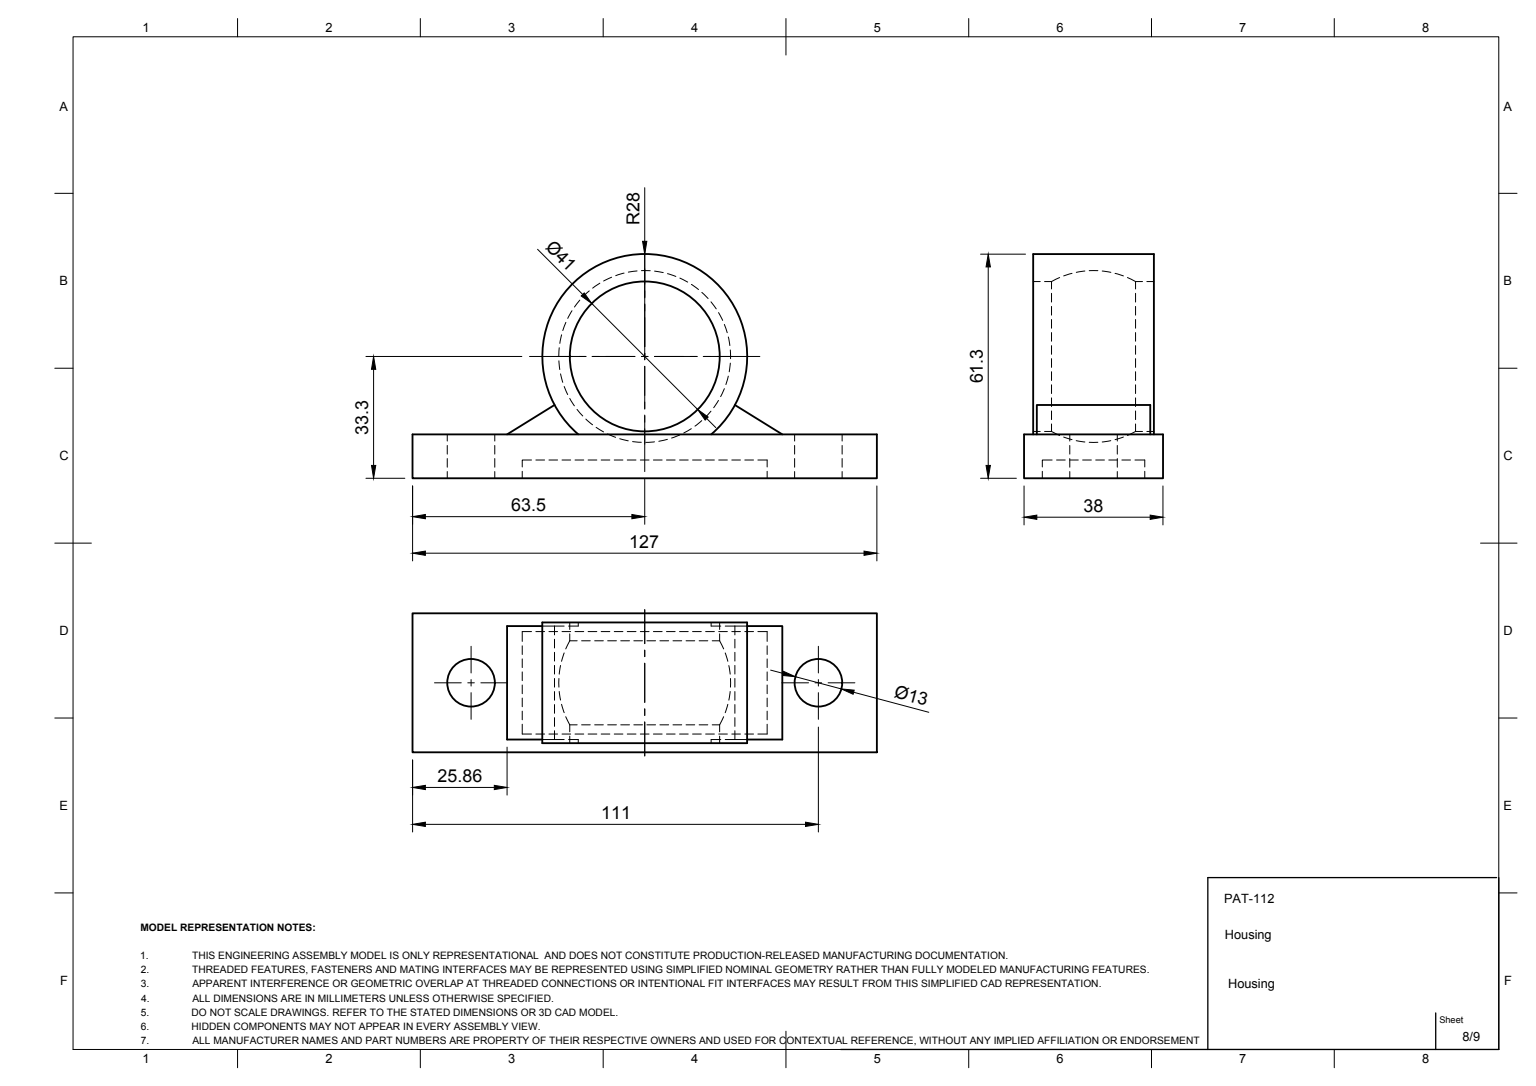
ISO-10303-21;
HEADER;
/* Generated by software containing ST-Developer
 * from STEP Tools, Inc. (www.steptools.com) 
 */

FILE_DESCRIPTION(
/* description */ ('PAT-112'),
/* implementation_level */ '2;1');

FILE_NAME(
/* name */ 'Housing.step',
/* time_stamp */ '2026-11-15T15:25:42-08:00',
/* author */ (''),
/* organization */ (''),
/* preprocessor_version */ 'ST-DEVELOPER v20.2',
/* originating_system */ 'Autodesk Translation Framework v15.17.0.0',
/* authorisation */ '');

FILE_SCHEMA (('AUTOMOTIVE_DESIGN { 1 0 10303 214 3 1 1 }'));
ENDSEC;

DATA;
#10=MECHANICAL_DESIGN_GEOMETRIC_PRESENTATION_REPRESENTATION('',(#106),#2277);
#89=SPHERICAL_SURFACE('',#1376,2.35);
#92=SHAPE_REPRESENTATION_RELATIONSHIP('SRR','None',#2321,#99);
#99=ADVANCED_BREP_SHAPE_REPRESENTATION('',(#114),#2271);
#106=STYLED_ITEM('',(#2368),#114);
#114=MANIFOLD_SOLID_BREP('Body1',#1258);
#124=FACE_BOUND('',#295,.T.);
#125=FACE_BOUND('',#296,.T.);
#126=FACE_BOUND('',#304,.T.);
#127=FACE_BOUND('',#305,.T.);
#128=FACE_BOUND('',#306,.T.);
#129=FACE_BOUND('',#309,.T.);
#130=FACE_BOUND('',#311,.T.);
#131=FACE_BOUND('',#324,.T.);
#132=FACE_BOUND('',#325,.T.);
#133=FACE_BOUND('',#326,.T.);
#156=PLANE('',#1378);
#157=PLANE('',#1380);
#158=PLANE('',#1382);
#159=PLANE('',#1384);
#160=PLANE('',#1385);
#161=PLANE('',#1387);
#162=PLANE('',#1388);
#163=PLANE('',#1394);
#164=PLANE('',#1395);
#165=PLANE('',#1396);
#166=PLANE('',#1397);
#167=PLANE('',#1398);
#168=PLANE('',#1399);
#169=PLANE('',#1400);
#170=PLANE('',#1405);
#171=PLANE('',#1406);
#172=PLANE('',#1407);
#173=PLANE('',#1408);
#174=PLANE('',#1409);
#211=FACE_OUTER_BOUND('',#292,.T.);
#212=FACE_OUTER_BOUND('',#293,.T.);
#213=FACE_OUTER_BOUND('',#294,.T.);
#214=FACE_OUTER_BOUND('',#297,.T.);
#215=FACE_OUTER_BOUND('',#298,.T.);
#216=FACE_OUTER_BOUND('',#299,.T.);
#217=FACE_OUTER_BOUND('',#300,.T.);
#218=FACE_OUTER_BOUND('',#301,.T.);
#219=FACE_OUTER_BOUND('',#302,.T.);
#220=FACE_OUTER_BOUND('',#303,.T.);
#221=FACE_OUTER_BOUND('',#307,.T.);
#222=FACE_OUTER_BOUND('',#308,.T.);
#223=FACE_OUTER_BOUND('',#310,.T.);
#224=FACE_OUTER_BOUND('',#312,.T.);
#225=FACE_OUTER_BOUND('',#313,.T.);
#226=FACE_OUTER_BOUND('',#314,.T.);
#227=FACE_OUTER_BOUND('',#315,.T.);
#228=FACE_OUTER_BOUND('',#316,.T.);
#229=FACE_OUTER_BOUND('',#317,.T.);
#230=FACE_OUTER_BOUND('',#318,.T.);
#231=FACE_OUTER_BOUND('',#319,.T.);
#232=FACE_OUTER_BOUND('',#320,.T.);
#233=FACE_OUTER_BOUND('',#321,.T.);
#234=FACE_OUTER_BOUND('',#322,.T.);
#235=FACE_OUTER_BOUND('',#323,.T.);
#292=EDGE_LOOP('',(#914,#915,#916,#917));
#293=EDGE_LOOP('',(#918,#919,#920,#921));
#294=EDGE_LOOP('',(#922,#923));
#295=EDGE_LOOP('',(#924));
#296=EDGE_LOOP('',(#925));
#297=EDGE_LOOP('',(#926,#927,#928));
#298=EDGE_LOOP('',(#929,#930,#931));
#299=EDGE_LOOP('',(#932,#933,#934));
#300=EDGE_LOOP('',(#935,#936,#937,#938));
#301=EDGE_LOOP('',(#939,#940,#941));
#302=EDGE_LOOP('',(#942,#943,#944,#945));
#303=EDGE_LOOP('',(#946,#947,#948,#949));
#304=EDGE_LOOP('',(#950));
#305=EDGE_LOOP('',(#951));
#306=EDGE_LOOP('',(#952,#953,#954,#955,#956,#957,#958,#959,#960,#961,#962,
#963));
#307=EDGE_LOOP('',(#964,#965,#966,#967,#968,#969,#970,#971,#972,#973,#974,
#975));
#308=EDGE_LOOP('',(#976,#977));
#309=EDGE_LOOP('',(#978));
#310=EDGE_LOOP('',(#979,#980));
#311=EDGE_LOOP('',(#981));
#312=EDGE_LOOP('',(#982,#983,#984,#985));
#313=EDGE_LOOP('',(#986,#987,#988,#989));
#314=EDGE_LOOP('',(#990,#991,#992,#993));
#315=EDGE_LOOP('',(#994,#995,#996,#997));
#316=EDGE_LOOP('',(#998,#999,#1000,#1001));
#317=EDGE_LOOP('',(#1002,#1003,#1004,#1005));
#318=EDGE_LOOP('',(#1006,#1007,#1008,#1009));
#319=EDGE_LOOP('',(#1010,#1011,#1012,#1013));
#320=EDGE_LOOP('',(#1014,#1015,#1016,#1017));
#321=EDGE_LOOP('',(#1018,#1019,#1020,#1021));
#322=EDGE_LOOP('',(#1022,#1023,#1024,#1025));
#323=EDGE_LOOP('',(#1026,#1027,#1028,#1029));
#324=EDGE_LOOP('',(#1030,#1031,#1032,#1033));
#325=EDGE_LOOP('',(#1034));
#326=EDGE_LOOP('',(#1035));
#393=LINE('',#1969,#488);
#394=LINE('',#1975,#489);
#395=LINE('',#1984,#490);
#396=LINE('',#1986,#491);
#397=LINE('',#1991,#492);
#398=LINE('',#1994,#493);
#399=LINE('',#1998,#494);
#400=LINE('',#2001,#495);
#401=LINE('',#2003,#496);
#402=LINE('',#2004,#497);
#403=LINE('',#2008,#498);
#404=LINE('',#2010,#499);
#405=LINE('',#2013,#500);
#406=LINE('',#2014,#501);
#407=LINE('',#2018,#502);
#408=LINE('',#2020,#503);
#409=LINE('',#2022,#504);
#410=LINE('',#2023,#505);
#411=LINE('',#2029,#506);
#412=LINE('',#2031,#507);
#413=LINE('',#2032,#508);
#414=LINE('',#2034,#509);
#415=LINE('',#2036,#510);
#416=LINE('',#2037,#511);
#417=LINE('',#2046,#512);
#418=LINE('',#2048,#513);
#419=LINE('',#2050,#514);
#420=LINE('',#2051,#515);
#421=LINE('',#2054,#516);
#422=LINE('',#2056,#517);
#423=LINE('',#2057,#518);
#424=LINE('',#2060,#519);
#425=LINE('',#2062,#520);
#426=LINE('',#2063,#521);
#427=LINE('',#2065,#522);
#428=LINE('',#2066,#523);
#429=LINE('',#2071,#524);
#430=LINE('',#2075,#525);
#431=LINE('',#2079,#526);
#432=LINE('',#2080,#527);
#433=LINE('',#2081,#528);
#434=LINE('',#2084,#529);
#435=LINE('',#2085,#530);
#436=LINE('',#2088,#531);
#437=LINE('',#2089,#532);
#438=LINE('',#2091,#533);
#488=VECTOR('',#1572,2.05);
#489=VECTOR('',#1579,2.05);
#490=VECTOR('',#1588,1.);
#491=VECTOR('',#1589,1.);
#492=VECTOR('',#1594,1.);
#493=VECTOR('',#1597,1.);
#494=VECTOR('',#1600,1.);
#495=VECTOR('',#1603,1.);
#496=VECTOR('',#1606,1.);
#497=VECTOR('',#1607,1.);
#498=VECTOR('',#1610,1.);
#499=VECTOR('',#1611,1.);
#500=VECTOR('',#1616,1.);
#501=VECTOR('',#1617,1.);
#502=VECTOR('',#1620,1.);
#503=VECTOR('',#1621,1.);
#504=VECTOR('',#1622,1.);
#505=VECTOR('',#1623,1.);
#506=VECTOR('',#1628,1.);
#507=VECTOR('',#1629,1.);
#508=VECTOR('',#1630,1.);
#509=VECTOR('',#1631,1.);
#510=VECTOR('',#1632,1.);
#511=VECTOR('',#1633,1.);
#512=VECTOR('',#1646,1.);
#513=VECTOR('',#1647,1.);
#514=VECTOR('',#1648,1.);
#515=VECTOR('',#1649,1.);
#516=VECTOR('',#1652,1.);
#517=VECTOR('',#1653,1.);
#518=VECTOR('',#1654,1.);
#519=VECTOR('',#1657,1.);
#520=VECTOR('',#1658,1.);
#521=VECTOR('',#1659,1.);
#522=VECTOR('',#1662,1.);
#523=VECTOR('',#1663,1.);
#524=VECTOR('',#1670,0.65);
#525=VECTOR('',#1675,0.65);
#526=VECTOR('',#1678,1.);
#527=VECTOR('',#1679,1.);
#528=VECTOR('',#1680,1.);
#529=VECTOR('',#1683,1.);
#530=VECTOR('',#1684,1.);
#531=VECTOR('',#1687,1.);
#532=VECTOR('',#1688,1.);
#533=VECTOR('',#1691,1.);
#575=CIRCLE('',#1371,2.05);
#576=CIRCLE('',#1372,2.05);
#577=CIRCLE('',#1374,2.05);
#578=CIRCLE('',#1375,2.05);
#579=CIRCLE('',#1377,2.35);
#580=CIRCLE('',#1379,2.8);
#581=CIRCLE('',#1381,2.8);
#582=CIRCLE('',#1383,2.8);
#583=CIRCLE('',#1386,2.8);
#584=CIRCLE('',#1389,0.65);
#585=CIRCLE('',#1390,0.65);
#586=CIRCLE('',#1392,2.8);
#587=CIRCLE('',#1393,2.8);
#588=CIRCLE('',#1402,0.65);
#589=CIRCLE('',#1404,0.65);
#635=VERTEX_POINT('',#1966);
#636=VERTEX_POINT('',#1968);
#637=VERTEX_POINT('',#1972);
#638=VERTEX_POINT('',#1974);
#639=VERTEX_POINT('',#1978);
#640=VERTEX_POINT('',#1979);
#641=VERTEX_POINT('',#1982);
#642=VERTEX_POINT('',#1983);
#643=VERTEX_POINT('',#1985);
#644=VERTEX_POINT('',#1989);
#645=VERTEX_POINT('',#1990);
#646=VERTEX_POINT('',#1992);
#647=VERTEX_POINT('',#1996);
#648=VERTEX_POINT('',#1997);
#649=VERTEX_POINT('',#1999);
#650=VERTEX_POINT('',#2006);
#651=VERTEX_POINT('',#2007);
#652=VERTEX_POINT('',#2009);
#653=VERTEX_POINT('',#2016);
#654=VERTEX_POINT('',#2017);
#655=VERTEX_POINT('',#2019);
#656=VERTEX_POINT('',#2021);
#657=VERTEX_POINT('',#2024);
#658=VERTEX_POINT('',#2026);
#659=VERTEX_POINT('',#2028);
#660=VERTEX_POINT('',#2030);
#661=VERTEX_POINT('',#2033);
#662=VERTEX_POINT('',#2035);
#663=VERTEX_POINT('',#2044);
#664=VERTEX_POINT('',#2045);
#665=VERTEX_POINT('',#2047);
#666=VERTEX_POINT('',#2049);
#667=VERTEX_POINT('',#2053);
#668=VERTEX_POINT('',#2055);
#669=VERTEX_POINT('',#2059);
#670=VERTEX_POINT('',#2061);
#671=VERTEX_POINT('',#2069);
#672=VERTEX_POINT('',#2073);
#673=VERTEX_POINT('',#2077);
#674=VERTEX_POINT('',#2078);
#675=VERTEX_POINT('',#2083);
#676=VERTEX_POINT('',#2087);
#743=EDGE_CURVE('',#635,#635,#575,.T.);
#744=EDGE_CURVE('',#635,#636,#393,.T.);
#745=EDGE_CURVE('',#636,#636,#576,.T.);
#746=EDGE_CURVE('',#637,#637,#577,.T.);
#747=EDGE_CURVE('',#637,#638,#394,.T.);
#748=EDGE_CURVE('',#638,#638,#578,.T.);
#749=EDGE_CURVE('',#639,#640,#579,.T.);
#750=EDGE_CURVE('',#641,#642,#395,.T.);
#751=EDGE_CURVE('',#641,#643,#396,.T.);
#752=EDGE_CURVE('',#642,#643,#580,.T.);
#753=EDGE_CURVE('',#644,#645,#397,.T.);
#754=EDGE_CURVE('',#646,#644,#581,.T.);
#755=EDGE_CURVE('',#646,#645,#398,.T.);
#756=EDGE_CURVE('',#647,#648,#399,.T.);
#757=EDGE_CURVE('',#649,#647,#582,.T.);
#758=EDGE_CURVE('',#649,#648,#400,.T.);
#759=EDGE_CURVE('',#648,#641,#401,.T.);
#760=EDGE_CURVE('',#643,#649,#402,.T.);
#761=EDGE_CURVE('',#650,#651,#403,.T.);
#762=EDGE_CURVE('',#650,#652,#404,.T.);
#763=EDGE_CURVE('',#651,#652,#583,.T.);
#764=EDGE_CURVE('',#645,#650,#405,.T.);
#765=EDGE_CURVE('',#652,#646,#406,.T.);
#766=EDGE_CURVE('',#653,#654,#407,.T.);
#767=EDGE_CURVE('',#654,#655,#408,.T.);
#768=EDGE_CURVE('',#655,#656,#409,.T.);
#769=EDGE_CURVE('',#656,#653,#410,.T.);
#770=EDGE_CURVE('',#657,#657,#584,.T.);
#771=EDGE_CURVE('',#658,#658,#585,.T.);
#772=EDGE_CURVE('',#651,#659,#411,.T.);
#773=EDGE_CURVE('',#659,#660,#412,.T.);
#774=EDGE_CURVE('',#660,#647,#413,.T.);
#775=EDGE_CURVE('',#642,#661,#414,.T.);
#776=EDGE_CURVE('',#661,#662,#415,.T.);
#777=EDGE_CURVE('',#662,#644,#416,.T.);
#778=EDGE_CURVE('',#661,#662,#586,.T.);
#779=EDGE_CURVE('',#659,#660,#587,.T.);
#780=EDGE_CURVE('',#663,#664,#417,.T.);
#781=EDGE_CURVE('',#663,#665,#418,.T.);
#782=EDGE_CURVE('',#665,#666,#419,.T.);
#783=EDGE_CURVE('',#664,#666,#420,.T.);
#784=EDGE_CURVE('',#667,#663,#421,.T.);
#785=EDGE_CURVE('',#667,#668,#422,.T.);
#786=EDGE_CURVE('',#668,#665,#423,.T.);
#787=EDGE_CURVE('',#669,#667,#424,.T.);
#788=EDGE_CURVE('',#669,#670,#425,.T.);
#789=EDGE_CURVE('',#670,#668,#426,.T.);
#790=EDGE_CURVE('',#664,#669,#427,.T.);
#791=EDGE_CURVE('',#666,#670,#428,.T.);
#792=EDGE_CURVE('',#671,#671,#588,.T.);
#793=EDGE_CURVE('',#671,#658,#429,.T.);
#794=EDGE_CURVE('',#672,#672,#589,.T.);
#795=EDGE_CURVE('',#672,#657,#430,.T.);
#796=EDGE_CURVE('',#673,#674,#431,.T.);
#797=EDGE_CURVE('',#674,#653,#432,.T.);
#798=EDGE_CURVE('',#673,#656,#433,.T.);
#799=EDGE_CURVE('',#675,#673,#434,.T.);
#800=EDGE_CURVE('',#675,#655,#435,.T.);
#801=EDGE_CURVE('',#676,#675,#436,.T.);
#802=EDGE_CURVE('',#676,#654,#437,.T.);
#803=EDGE_CURVE('',#674,#676,#438,.T.);
#914=ORIENTED_EDGE('',*,*,#743,.F.);
#915=ORIENTED_EDGE('',*,*,#744,.T.);
#916=ORIENTED_EDGE('',*,*,#745,.F.);
#917=ORIENTED_EDGE('',*,*,#744,.F.);
#918=ORIENTED_EDGE('',*,*,#746,.F.);
#919=ORIENTED_EDGE('',*,*,#747,.T.);
#920=ORIENTED_EDGE('',*,*,#748,.F.);
#921=ORIENTED_EDGE('',*,*,#747,.F.);
#922=ORIENTED_EDGE('',*,*,#749,.T.);
#923=ORIENTED_EDGE('',*,*,#749,.F.);
#924=ORIENTED_EDGE('',*,*,#746,.T.);
#925=ORIENTED_EDGE('',*,*,#745,.T.);
#926=ORIENTED_EDGE('',*,*,#750,.F.);
#927=ORIENTED_EDGE('',*,*,#751,.T.);
#928=ORIENTED_EDGE('',*,*,#752,.F.);
#929=ORIENTED_EDGE('',*,*,#753,.F.);
#930=ORIENTED_EDGE('',*,*,#754,.F.);
#931=ORIENTED_EDGE('',*,*,#755,.T.);
#932=ORIENTED_EDGE('',*,*,#756,.F.);
#933=ORIENTED_EDGE('',*,*,#757,.F.);
#934=ORIENTED_EDGE('',*,*,#758,.T.);
#935=ORIENTED_EDGE('',*,*,#759,.F.);
#936=ORIENTED_EDGE('',*,*,#758,.F.);
#937=ORIENTED_EDGE('',*,*,#760,.F.);
#938=ORIENTED_EDGE('',*,*,#751,.F.);
#939=ORIENTED_EDGE('',*,*,#761,.F.);
#940=ORIENTED_EDGE('',*,*,#762,.T.);
#941=ORIENTED_EDGE('',*,*,#763,.F.);
#942=ORIENTED_EDGE('',*,*,#764,.F.);
#943=ORIENTED_EDGE('',*,*,#755,.F.);
#944=ORIENTED_EDGE('',*,*,#765,.F.);
#945=ORIENTED_EDGE('',*,*,#762,.F.);
#946=ORIENTED_EDGE('',*,*,#766,.T.);
#947=ORIENTED_EDGE('',*,*,#767,.T.);
#948=ORIENTED_EDGE('',*,*,#768,.T.);
#949=ORIENTED_EDGE('',*,*,#769,.T.);
#950=ORIENTED_EDGE('',*,*,#770,.T.);
#951=ORIENTED_EDGE('',*,*,#771,.T.);
#952=ORIENTED_EDGE('',*,*,#753,.T.);
#953=ORIENTED_EDGE('',*,*,#764,.T.);
#954=ORIENTED_EDGE('',*,*,#761,.T.);
#955=ORIENTED_EDGE('',*,*,#772,.T.);
#956=ORIENTED_EDGE('',*,*,#773,.T.);
#957=ORIENTED_EDGE('',*,*,#774,.T.);
#958=ORIENTED_EDGE('',*,*,#756,.T.);
#959=ORIENTED_EDGE('',*,*,#759,.T.);
#960=ORIENTED_EDGE('',*,*,#750,.T.);
#961=ORIENTED_EDGE('',*,*,#775,.T.);
#962=ORIENTED_EDGE('',*,*,#776,.T.);
#963=ORIENTED_EDGE('',*,*,#777,.T.);
#964=ORIENTED_EDGE('',*,*,#754,.T.);
#965=ORIENTED_EDGE('',*,*,#777,.F.);
#966=ORIENTED_EDGE('',*,*,#778,.F.);
#967=ORIENTED_EDGE('',*,*,#775,.F.);
#968=ORIENTED_EDGE('',*,*,#752,.T.);
#969=ORIENTED_EDGE('',*,*,#760,.T.);
#970=ORIENTED_EDGE('',*,*,#757,.T.);
#971=ORIENTED_EDGE('',*,*,#774,.F.);
#972=ORIENTED_EDGE('',*,*,#779,.F.);
#973=ORIENTED_EDGE('',*,*,#772,.F.);
#974=ORIENTED_EDGE('',*,*,#763,.T.);
#975=ORIENTED_EDGE('',*,*,#765,.T.);
#976=ORIENTED_EDGE('',*,*,#773,.F.);
#977=ORIENTED_EDGE('',*,*,#779,.T.);
#978=ORIENTED_EDGE('',*,*,#743,.T.);
#979=ORIENTED_EDGE('',*,*,#776,.F.);
#980=ORIENTED_EDGE('',*,*,#778,.T.);
#981=ORIENTED_EDGE('',*,*,#748,.T.);
#982=ORIENTED_EDGE('',*,*,#780,.F.);
#983=ORIENTED_EDGE('',*,*,#781,.T.);
#984=ORIENTED_EDGE('',*,*,#782,.T.);
#985=ORIENTED_EDGE('',*,*,#783,.F.);
#986=ORIENTED_EDGE('',*,*,#784,.F.);
#987=ORIENTED_EDGE('',*,*,#785,.T.);
#988=ORIENTED_EDGE('',*,*,#786,.T.);
#989=ORIENTED_EDGE('',*,*,#781,.F.);
#990=ORIENTED_EDGE('',*,*,#787,.F.);
#991=ORIENTED_EDGE('',*,*,#788,.T.);
#992=ORIENTED_EDGE('',*,*,#789,.T.);
#993=ORIENTED_EDGE('',*,*,#785,.F.);
#994=ORIENTED_EDGE('',*,*,#790,.F.);
#995=ORIENTED_EDGE('',*,*,#783,.T.);
#996=ORIENTED_EDGE('',*,*,#791,.T.);
#997=ORIENTED_EDGE('',*,*,#788,.F.);
#998=ORIENTED_EDGE('',*,*,#791,.F.);
#999=ORIENTED_EDGE('',*,*,#782,.F.);
#1000=ORIENTED_EDGE('',*,*,#786,.F.);
#1001=ORIENTED_EDGE('',*,*,#789,.F.);
#1002=ORIENTED_EDGE('',*,*,#792,.F.);
#1003=ORIENTED_EDGE('',*,*,#793,.T.);
#1004=ORIENTED_EDGE('',*,*,#771,.F.);
#1005=ORIENTED_EDGE('',*,*,#793,.F.);
#1006=ORIENTED_EDGE('',*,*,#794,.F.);
#1007=ORIENTED_EDGE('',*,*,#795,.T.);
#1008=ORIENTED_EDGE('',*,*,#770,.F.);
#1009=ORIENTED_EDGE('',*,*,#795,.F.);
#1010=ORIENTED_EDGE('',*,*,#796,.T.);
#1011=ORIENTED_EDGE('',*,*,#797,.T.);
#1012=ORIENTED_EDGE('',*,*,#769,.F.);
#1013=ORIENTED_EDGE('',*,*,#798,.F.);
#1014=ORIENTED_EDGE('',*,*,#799,.T.);
#1015=ORIENTED_EDGE('',*,*,#798,.T.);
#1016=ORIENTED_EDGE('',*,*,#768,.F.);
#1017=ORIENTED_EDGE('',*,*,#800,.F.);
#1018=ORIENTED_EDGE('',*,*,#801,.T.);
#1019=ORIENTED_EDGE('',*,*,#800,.T.);
#1020=ORIENTED_EDGE('',*,*,#767,.F.);
#1021=ORIENTED_EDGE('',*,*,#802,.F.);
#1022=ORIENTED_EDGE('',*,*,#803,.T.);
#1023=ORIENTED_EDGE('',*,*,#802,.T.);
#1024=ORIENTED_EDGE('',*,*,#766,.F.);
#1025=ORIENTED_EDGE('',*,*,#797,.F.);
#1026=ORIENTED_EDGE('',*,*,#803,.F.);
#1027=ORIENTED_EDGE('',*,*,#796,.F.);
#1028=ORIENTED_EDGE('',*,*,#799,.F.);
#1029=ORIENTED_EDGE('',*,*,#801,.F.);
#1030=ORIENTED_EDGE('',*,*,#780,.T.);
#1031=ORIENTED_EDGE('',*,*,#790,.T.);
#1032=ORIENTED_EDGE('',*,*,#787,.T.);
#1033=ORIENTED_EDGE('',*,*,#784,.T.);
#1034=ORIENTED_EDGE('',*,*,#792,.T.);
#1035=ORIENTED_EDGE('',*,*,#794,.T.);
#1164=CYLINDRICAL_SURFACE('',#1370,2.05);
#1165=CYLINDRICAL_SURFACE('',#1373,2.05);
#1166=CYLINDRICAL_SURFACE('',#1391,2.8);
#1167=CYLINDRICAL_SURFACE('',#1401,0.65);
#1168=CYLINDRICAL_SURFACE('',#1403,0.65);
#1194=ADVANCED_FACE('',(#211),#1164,.F.);
#1195=ADVANCED_FACE('',(#212),#1165,.F.);
#1196=ADVANCED_FACE('',(#213,#124,#125),#89,.F.);
#1197=ADVANCED_FACE('',(#214),#156,.T.);
#1198=ADVANCED_FACE('',(#215),#157,.T.);
#1199=ADVANCED_FACE('',(#216),#158,.T.);
#1200=ADVANCED_FACE('',(#217),#159,.T.);
#1201=ADVANCED_FACE('',(#218),#160,.T.);
#1202=ADVANCED_FACE('',(#219),#161,.T.);
#1203=ADVANCED_FACE('',(#220,#126,#127,#128),#162,.T.);
#1204=ADVANCED_FACE('',(#221),#1166,.T.);
#1205=ADVANCED_FACE('',(#222,#129),#163,.F.);
#1206=ADVANCED_FACE('',(#223,#130),#164,.T.);
#1207=ADVANCED_FACE('',(#224),#165,.F.);
#1208=ADVANCED_FACE('',(#225),#166,.F.);
#1209=ADVANCED_FACE('',(#226),#167,.F.);
#1210=ADVANCED_FACE('',(#227),#168,.F.);
#1211=ADVANCED_FACE('',(#228),#169,.F.);
#1212=ADVANCED_FACE('',(#229),#1167,.F.);
#1213=ADVANCED_FACE('',(#230),#1168,.F.);
#1214=ADVANCED_FACE('',(#231),#170,.T.);
#1215=ADVANCED_FACE('',(#232),#171,.T.);
#1216=ADVANCED_FACE('',(#233),#172,.T.);
#1217=ADVANCED_FACE('',(#234),#173,.T.);
#1218=ADVANCED_FACE('',(#235,#131,#132,#133),#174,.F.);
#1258=CLOSED_SHELL('',(#1194,#1195,#1196,#1197,#1198,#1199,#1200,#1201,
#1202,#1203,#1204,#1205,#1206,#1207,#1208,#1209,#1210,#1211,#1212,#1213,
#1214,#1215,#1216,#1217,#1218));
#1369=AXIS2_PLACEMENT_3D('',#1964,#1566,#1567);
#1370=AXIS2_PLACEMENT_3D('',#1965,#1568,#1569);
#1371=AXIS2_PLACEMENT_3D('',#1967,#1570,#1571);
#1372=AXIS2_PLACEMENT_3D('',#1970,#1573,#1574);
#1373=AXIS2_PLACEMENT_3D('',#1971,#1575,#1576);
#1374=AXIS2_PLACEMENT_3D('',#1973,#1577,#1578);
#1375=AXIS2_PLACEMENT_3D('',#1976,#1580,#1581);
#1376=AXIS2_PLACEMENT_3D('',#1977,#1582,#1583);
#1377=AXIS2_PLACEMENT_3D('',#1980,#1584,#1585);
#1378=AXIS2_PLACEMENT_3D('',#1981,#1586,#1587);
#1379=AXIS2_PLACEMENT_3D('',#1987,#1590,#1591);
#1380=AXIS2_PLACEMENT_3D('',#1988,#1592,#1593);
#1381=AXIS2_PLACEMENT_3D('',#1993,#1595,#1596);
#1382=AXIS2_PLACEMENT_3D('',#1995,#1598,#1599);
#1383=AXIS2_PLACEMENT_3D('',#2000,#1601,#1602);
#1384=AXIS2_PLACEMENT_3D('',#2002,#1604,#1605);
#1385=AXIS2_PLACEMENT_3D('',#2005,#1608,#1609);
#1386=AXIS2_PLACEMENT_3D('',#2011,#1612,#1613);
#1387=AXIS2_PLACEMENT_3D('',#2012,#1614,#1615);
#1388=AXIS2_PLACEMENT_3D('',#2015,#1618,#1619);
#1389=AXIS2_PLACEMENT_3D('',#2025,#1624,#1625);
#1390=AXIS2_PLACEMENT_3D('',#2027,#1626,#1627);
#1391=AXIS2_PLACEMENT_3D('',#2038,#1634,#1635);
#1392=AXIS2_PLACEMENT_3D('',#2039,#1636,#1637);
#1393=AXIS2_PLACEMENT_3D('',#2040,#1638,#1639);
#1394=AXIS2_PLACEMENT_3D('',#2041,#1640,#1641);
#1395=AXIS2_PLACEMENT_3D('',#2042,#1642,#1643);
#1396=AXIS2_PLACEMENT_3D('',#2043,#1644,#1645);
#1397=AXIS2_PLACEMENT_3D('',#2052,#1650,#1651);
#1398=AXIS2_PLACEMENT_3D('',#2058,#1655,#1656);
#1399=AXIS2_PLACEMENT_3D('',#2064,#1660,#1661);
#1400=AXIS2_PLACEMENT_3D('',#2067,#1664,#1665);
#1401=AXIS2_PLACEMENT_3D('',#2068,#1666,#1667);
#1402=AXIS2_PLACEMENT_3D('',#2070,#1668,#1669);
#1403=AXIS2_PLACEMENT_3D('',#2072,#1671,#1672);
#1404=AXIS2_PLACEMENT_3D('',#2074,#1673,#1674);
#1405=AXIS2_PLACEMENT_3D('',#2076,#1676,#1677);
#1406=AXIS2_PLACEMENT_3D('',#2082,#1681,#1682);
#1407=AXIS2_PLACEMENT_3D('',#2086,#1685,#1686);
#1408=AXIS2_PLACEMENT_3D('',#2090,#1689,#1690);
#1409=AXIS2_PLACEMENT_3D('',#2092,#1692,#1693);
#1566=DIRECTION('axis',(0.,0.,1.));
#1567=DIRECTION('refdir',(1.,0.,0.));
#1568=DIRECTION('center_axis',(0.,1.,0.));
#1569=DIRECTION('ref_axis',(1.,0.,0.));
#1570=DIRECTION('center_axis',(0.,1.,0.));
#1571=DIRECTION('ref_axis',(1.,0.,0.));
#1572=DIRECTION('',(0.,1.,0.));
#1573=DIRECTION('center_axis',(0.,-1.,0.));
#1574=DIRECTION('ref_axis',(1.,0.,0.));
#1575=DIRECTION('center_axis',(0.,1.,0.));
#1576=DIRECTION('ref_axis',(1.,0.,0.));
#1577=DIRECTION('center_axis',(0.,1.,0.));
#1578=DIRECTION('ref_axis',(1.,0.,0.));
#1579=DIRECTION('',(0.,1.,0.));
#1580=DIRECTION('center_axis',(0.,-1.,0.));
#1581=DIRECTION('ref_axis',(1.,0.,0.));
#1582=DIRECTION('center_axis',(1.22464679914735E-16,0.,1.));
#1583=DIRECTION('ref_axis',(1.,0.,-6.12323399573677E-17));
#1584=DIRECTION('center_axis',(-1.22464679914735E-16,1.,7.49879891330929E-33));
#1585=DIRECTION('ref_axis',(-1.,-1.22464679914735E-16,6.12323399573677E-17));
#1586=DIRECTION('center_axis',(0.,1.,0.));
#1587=DIRECTION('ref_axis',(0.,0.,1.));
#1588=DIRECTION('',(1.,0.,0.));
#1589=DIRECTION('',(0.850265146687862,0.,0.526354614616295));
#1590=DIRECTION('center_axis',(0.,1.,0.));
#1591=DIRECTION('ref_axis',(1.,0.,0.));
#1592=DIRECTION('center_axis',(0.,1.,0.));
#1593=DIRECTION('ref_axis',(0.,0.,1.));
#1594=DIRECTION('',(1.,0.,0.));
#1595=DIRECTION('center_axis',(0.,1.,0.));
#1596=DIRECTION('ref_axis',(1.,0.,0.));
#1597=DIRECTION('',(0.850265146687862,0.,-0.526354614616295));
#1598=DIRECTION('center_axis',(0.,-1.,0.));
#1599=DIRECTION('ref_axis',(0.,0.,-1.));
#1600=DIRECTION('',(-1.,0.,0.));
#1601=DIRECTION('center_axis',(0.,-1.,0.));
#1602=DIRECTION('ref_axis',(1.,0.,0.));
#1603=DIRECTION('',(-0.850265146687862,0.,-0.526354614616295));
#1604=DIRECTION('center_axis',(-0.526354614616295,0.,0.850265146687862));
#1605=DIRECTION('ref_axis',(0.850265146687862,0.,0.526354614616295));
#1606=DIRECTION('',(0.,1.,0.));
#1607=DIRECTION('',(0.,-1.,0.));
#1608=DIRECTION('center_axis',(0.,-1.,0.));
#1609=DIRECTION('ref_axis',(0.,0.,-1.));
#1610=DIRECTION('',(-1.,0.,0.));
#1611=DIRECTION('',(-0.850265146687862,0.,0.526354614616295));
#1612=DIRECTION('center_axis',(0.,-1.,0.));
#1613=DIRECTION('ref_axis',(1.,0.,0.));
#1614=DIRECTION('center_axis',(0.526354614616295,0.,0.850265146687862));
#1615=DIRECTION('ref_axis',(0.850265146687862,0.,-0.526354614616295));
#1616=DIRECTION('',(0.,-1.,0.));
#1617=DIRECTION('',(0.,1.,0.));
#1618=DIRECTION('center_axis',(0.,0.,1.));
#1619=DIRECTION('ref_axis',(1.,0.,0.));
#1620=DIRECTION('',(0.,-1.,0.));
#1621=DIRECTION('',(1.,0.,0.));
#1622=DIRECTION('',(0.,1.,0.));
#1623=DIRECTION('',(-1.,0.,0.));
#1624=DIRECTION('center_axis',(0.,0.,-1.));
#1625=DIRECTION('ref_axis',(1.,0.,0.));
#1626=DIRECTION('center_axis',(0.,0.,-1.));
#1627=DIRECTION('ref_axis',(1.,0.,0.));
#1628=DIRECTION('',(0.,-1.,0.));
#1629=DIRECTION('',(-1.,0.,0.));
#1630=DIRECTION('',(0.,1.,0.));
#1631=DIRECTION('',(0.,1.,0.));
#1632=DIRECTION('',(1.,0.,0.));
#1633=DIRECTION('',(0.,-1.,0.));
#1634=DIRECTION('center_axis',(0.,1.,0.));
#1635=DIRECTION('ref_axis',(6.12323399573677E-17,0.,1.));
#1636=DIRECTION('center_axis',(0.,1.,0.));
#1637=DIRECTION('ref_axis',(1.,0.,0.));
#1638=DIRECTION('center_axis',(0.,-1.,0.));
#1639=DIRECTION('ref_axis',(1.,0.,0.));
#1640=DIRECTION('center_axis',(0.,1.,0.));
#1641=DIRECTION('ref_axis',(1.,0.,0.));
#1642=DIRECTION('center_axis',(0.,1.,0.));
#1643=DIRECTION('ref_axis',(1.,0.,0.));
#1644=DIRECTION('center_axis',(0.,1.,0.));
#1645=DIRECTION('ref_axis',(-1.,0.,0.));
#1646=DIRECTION('',(-1.,0.,0.));
#1647=DIRECTION('',(0.,0.,1.));
#1648=DIRECTION('',(-1.,0.,0.));
#1649=DIRECTION('',(0.,0.,1.));
#1650=DIRECTION('center_axis',(1.,0.,0.));
#1651=DIRECTION('ref_axis',(0.,1.,0.));
#1652=DIRECTION('',(0.,1.,0.));
#1653=DIRECTION('',(0.,0.,1.));
#1654=DIRECTION('',(0.,1.,0.));
#1655=DIRECTION('center_axis',(0.,-1.,0.));
#1656=DIRECTION('ref_axis',(1.,0.,0.));
#1657=DIRECTION('',(1.,0.,0.));
#1658=DIRECTION('',(0.,0.,1.));
#1659=DIRECTION('',(1.,0.,0.));
#1660=DIRECTION('center_axis',(-1.,0.,0.));
#1661=DIRECTION('ref_axis',(0.,-1.,0.));
#1662=DIRECTION('',(0.,-1.,0.));
#1663=DIRECTION('',(0.,-1.,0.));
#1664=DIRECTION('center_axis',(0.,0.,1.));
#1665=DIRECTION('ref_axis',(1.,0.,0.));
#1666=DIRECTION('center_axis',(0.,0.,1.));
#1667=DIRECTION('ref_axis',(1.,0.,0.));
#1668=DIRECTION('center_axis',(0.,0.,1.));
#1669=DIRECTION('ref_axis',(1.,0.,0.));
#1670=DIRECTION('',(0.,0.,1.));
#1671=DIRECTION('center_axis',(0.,0.,1.));
#1672=DIRECTION('ref_axis',(1.,0.,0.));
#1673=DIRECTION('center_axis',(0.,0.,1.));
#1674=DIRECTION('ref_axis',(1.,0.,0.));
#1675=DIRECTION('',(0.,0.,1.));
#1676=DIRECTION('center_axis',(0.,1.,0.));
#1677=DIRECTION('ref_axis',(-1.,0.,0.));
#1678=DIRECTION('',(-1.,0.,0.));
#1679=DIRECTION('',(0.,0.,1.));
#1680=DIRECTION('',(0.,0.,1.));
#1681=DIRECTION('center_axis',(1.,0.,0.));
#1682=DIRECTION('ref_axis',(0.,1.,0.));
#1683=DIRECTION('',(0.,1.,0.));
#1684=DIRECTION('',(0.,0.,1.));
#1685=DIRECTION('center_axis',(0.,-1.,0.));
#1686=DIRECTION('ref_axis',(1.,0.,0.));
#1687=DIRECTION('',(1.,0.,0.));
#1688=DIRECTION('',(0.,0.,1.));
#1689=DIRECTION('center_axis',(-1.,0.,0.));
#1690=DIRECTION('ref_axis',(0.,-1.,0.));
#1691=DIRECTION('',(0.,-1.,0.));
#1692=DIRECTION('center_axis',(0.,0.,1.));
#1693=DIRECTION('ref_axis',(1.,0.,0.));
#1964=CARTESIAN_POINT('',(0.,0.,0.));
#1965=CARTESIAN_POINT('Origin',(0.,0.,0.));
#1966=CARTESIAN_POINT('',(-2.05,-1.65,2.51052593825207E-16));
#1967=CARTESIAN_POINT('Origin',(0.,-1.65,0.));
#1968=CARTESIAN_POINT('',(-2.05,-1.14891252930761,-2.51052593825207E-16));
#1969=CARTESIAN_POINT('',(-2.05,0.,2.51052593825207E-16));
#1970=CARTESIAN_POINT('Origin',(0.,-1.14891252930761,0.));
#1971=CARTESIAN_POINT('Origin',(0.,0.,0.));
#1972=CARTESIAN_POINT('',(-2.05,1.14891252930761,2.51052593825207E-16));
#1973=CARTESIAN_POINT('Origin',(0.,1.14891252930761,0.));
#1974=CARTESIAN_POINT('',(-2.05,1.65,-2.51052593825207E-16));
#1975=CARTESIAN_POINT('',(-2.05,0.,2.51052593825207E-16));
#1976=CARTESIAN_POINT('Origin',(0.,1.65,0.));
#1977=CARTESIAN_POINT('Origin',(0.,0.,0.));
#1978=CARTESIAN_POINT('',(-2.87791997799628E-16,-1.76221774462768E-32,-2.35));
#1979=CARTESIAN_POINT('',(7.39557098644699E-32,-1.76221774462768E-32,2.35));
#1980=CARTESIAN_POINT('Origin',(0.,0.,0.));
#1981=CARTESIAN_POINT('Origin',(0.,1.55,-1.49));
#1982=CARTESIAN_POINT('',(-3.76384615384615,1.55,-2.13));
#1983=CARTESIAN_POINT('',(-1.81744325908679,1.55,-2.13));
#1984=CARTESIAN_POINT('',(0.,1.55,-2.13));
#1985=CARTESIAN_POINT('',(-2.46585583768694,1.55,-1.32648218523477));
#1986=CARTESIAN_POINT('',(-1.68,1.55,-0.84));
#1987=CARTESIAN_POINT('Origin',(0.,1.55,0.));
#1988=CARTESIAN_POINT('Origin',(0.,1.55,-1.49));
#1989=CARTESIAN_POINT('',(1.81744325908679,1.55,-2.13));
#1990=CARTESIAN_POINT('',(3.76384615384615,1.55,-2.13));
#1991=CARTESIAN_POINT('',(0.,1.55,-2.13));
#1992=CARTESIAN_POINT('',(2.46585583768694,1.55,-1.32648218523477));
#1993=CARTESIAN_POINT('Origin',(0.,1.55,0.));
#1994=CARTESIAN_POINT('',(3.78,1.55,-2.14));
#1995=CARTESIAN_POINT('Origin',(0.,-1.55,-1.49));
#1996=CARTESIAN_POINT('',(-1.81744325908679,-1.55,-2.13));
#1997=CARTESIAN_POINT('',(-3.76384615384615,-1.55,-2.13));
#1998=CARTESIAN_POINT('',(0.,-1.55,-2.13));
#1999=CARTESIAN_POINT('',(-2.46585583768694,-1.55,-1.32648218523477));
#2000=CARTESIAN_POINT('Origin',(0.,-1.55,0.));
#2001=CARTESIAN_POINT('',(-1.68,-1.55,-0.84));
#2002=CARTESIAN_POINT('Origin',(-3.78,0.,-2.14));
#2003=CARTESIAN_POINT('',(-3.76384615384615,0.,-2.13));
#2004=CARTESIAN_POINT('',(-2.46585583768694,0.,-1.32648218523477));
#2005=CARTESIAN_POINT('Origin',(0.,-1.55,-1.49));
#2006=CARTESIAN_POINT('',(3.76384615384615,-1.55,-2.13));
#2007=CARTESIAN_POINT('',(1.81744325908679,-1.55,-2.13));
#2008=CARTESIAN_POINT('',(0.,-1.55,-2.13));
#2009=CARTESIAN_POINT('',(2.46585583768694,-1.55,-1.32648218523477));
#2010=CARTESIAN_POINT('',(3.78,-1.55,-2.14));
#2011=CARTESIAN_POINT('Origin',(0.,-1.55,0.));
#2012=CARTESIAN_POINT('Origin',(1.68,0.,-0.84));
#2013=CARTESIAN_POINT('',(3.76384615384615,0.,-2.13));
#2014=CARTESIAN_POINT('',(2.46585583768694,0.,-1.32648218523477));
#2015=CARTESIAN_POINT('Origin',(0.,0.,-2.13));
#2016=CARTESIAN_POINT('',(-6.35,1.9,-2.13));
#2017=CARTESIAN_POINT('',(-6.35,-1.9,-2.13));
#2018=CARTESIAN_POINT('',(-6.35,1.9,-2.13));
#2019=CARTESIAN_POINT('',(6.35,-1.9,-2.13));
#2020=CARTESIAN_POINT('',(-6.35,-1.9,-2.13));
#2021=CARTESIAN_POINT('',(6.35,1.9,-2.13));
#2022=CARTESIAN_POINT('',(6.35,-1.9,-2.13));
#2023=CARTESIAN_POINT('',(6.35,1.9,-2.13));
#2024=CARTESIAN_POINT('',(4.1,7.9602041944578E-17,-2.13));
#2025=CARTESIAN_POINT('Origin',(4.75,0.,-2.13));
#2026=CARTESIAN_POINT('',(-5.4,7.9602041944578E-17,-2.13));
#2027=CARTESIAN_POINT('Origin',(-4.75,0.,-2.13));
#2028=CARTESIAN_POINT('',(1.81744325908679,-1.65,-2.13));
#2029=CARTESIAN_POINT('',(1.81744325908679,0.,-2.13));
#2030=CARTESIAN_POINT('',(-1.81744325908679,-1.65,-2.13));
#2031=CARTESIAN_POINT('',(0.,-1.65,-2.13));
#2032=CARTESIAN_POINT('',(-1.81744325908679,0.,-2.13));
#2033=CARTESIAN_POINT('',(-1.81744325908679,1.65,-2.13));
#2034=CARTESIAN_POINT('',(-1.81744325908679,0.,-2.13));
#2035=CARTESIAN_POINT('',(1.81744325908679,1.65,-2.13));
#2036=CARTESIAN_POINT('',(0.,1.65,-2.13));
#2037=CARTESIAN_POINT('',(1.81744325908679,0.,-2.13));
#2038=CARTESIAN_POINT('Origin',(0.,0.,0.));
#2039=CARTESIAN_POINT('Origin',(0.,1.65,0.));
#2040=CARTESIAN_POINT('Origin',(0.,-1.65,0.));
#2041=CARTESIAN_POINT('Origin',(0.,-1.65,0.));
#2042=CARTESIAN_POINT('Origin',(0.,1.65,0.));
#2043=CARTESIAN_POINT('Origin',(3.35,1.4,-3.33));
#2044=CARTESIAN_POINT('',(3.35,1.4,-3.33));
#2045=CARTESIAN_POINT('',(-3.35,1.4,-3.33));
#2046=CARTESIAN_POINT('',(1.675,1.4,-3.33));
#2047=CARTESIAN_POINT('',(3.35,1.4,-2.83));
#2048=CARTESIAN_POINT('',(3.35,1.4,-3.33));
#2049=CARTESIAN_POINT('',(-3.35,1.4,-2.83));
#2050=CARTESIAN_POINT('',(3.35,1.4,-2.83));
#2051=CARTESIAN_POINT('',(-3.35,1.4,-3.33));
#2052=CARTESIAN_POINT('Origin',(3.35,-1.4,-3.33));
#2053=CARTESIAN_POINT('',(3.35,-1.4,-3.33));
#2054=CARTESIAN_POINT('',(3.35,-0.7,-3.33));
#2055=CARTESIAN_POINT('',(3.35,-1.4,-2.83));
#2056=CARTESIAN_POINT('',(3.35,-1.4,-3.33));
#2057=CARTESIAN_POINT('',(3.35,-1.4,-2.83));
#2058=CARTESIAN_POINT('Origin',(-3.35,-1.4,-3.33));
#2059=CARTESIAN_POINT('',(-3.35,-1.4,-3.33));
#2060=CARTESIAN_POINT('',(-1.675,-1.4,-3.33));
#2061=CARTESIAN_POINT('',(-3.35,-1.4,-2.83));
#2062=CARTESIAN_POINT('',(-3.35,-1.4,-3.33));
#2063=CARTESIAN_POINT('',(-3.35,-1.4,-2.83));
#2064=CARTESIAN_POINT('Origin',(-3.35,1.4,-3.33));
#2065=CARTESIAN_POINT('',(-3.35,0.7,-3.33));
#2066=CARTESIAN_POINT('',(-3.35,1.4,-2.83));
#2067=CARTESIAN_POINT('Origin',(0.,0.,-2.83));
#2068=CARTESIAN_POINT('Origin',(-4.75,0.,-3.33));
#2069=CARTESIAN_POINT('',(-5.4,-7.9602041944578E-17,-3.33));
#2070=CARTESIAN_POINT('Origin',(-4.75,0.,-3.33));
#2071=CARTESIAN_POINT('',(-5.4,-7.9602041944578E-17,-3.33));
#2072=CARTESIAN_POINT('Origin',(4.75,0.,-3.33));
#2073=CARTESIAN_POINT('',(4.1,-7.9602041944578E-17,-3.33));
#2074=CARTESIAN_POINT('Origin',(4.75,0.,-3.33));
#2075=CARTESIAN_POINT('',(4.1,-7.9602041944578E-17,-3.33));
#2076=CARTESIAN_POINT('Origin',(6.35,1.9,-3.33));
#2077=CARTESIAN_POINT('',(6.35,1.9,-3.33));
#2078=CARTESIAN_POINT('',(-6.35,1.9,-3.33));
#2079=CARTESIAN_POINT('',(6.35,1.9,-3.33));
#2080=CARTESIAN_POINT('',(-6.35,1.9,-3.33));
#2081=CARTESIAN_POINT('',(6.35,1.9,-3.33));
#2082=CARTESIAN_POINT('Origin',(6.35,-1.9,-3.33));
#2083=CARTESIAN_POINT('',(6.35,-1.9,-3.33));
#2084=CARTESIAN_POINT('',(6.35,-1.9,-3.33));
#2085=CARTESIAN_POINT('',(6.35,-1.9,-3.33));
#2086=CARTESIAN_POINT('Origin',(-6.35,-1.9,-3.33));
#2087=CARTESIAN_POINT('',(-6.35,-1.9,-3.33));
#2088=CARTESIAN_POINT('',(-6.35,-1.9,-3.33));
#2089=CARTESIAN_POINT('',(-6.35,-1.9,-3.33));
#2090=CARTESIAN_POINT('Origin',(-6.35,1.9,-3.33));
#2091=CARTESIAN_POINT('',(-6.35,1.9,-3.33));
#2092=CARTESIAN_POINT('Origin',(0.,0.,-3.33));
#2261=UNCERTAINTY_MEASURE_WITH_UNIT(LENGTH_MEASURE(0.001),#2278,
'DISTANCE_ACCURACY_VALUE',
'Maximum model space distance between geometric entities at asserted c
onnectivities');
#2267=UNCERTAINTY_MEASURE_WITH_UNIT(LENGTH_MEASURE(0.001),#2278,
'DISTANCE_ACCURACY_VALUE',
'Maximum model space distance between geometric entities at asserted c
onnectivities');
#2271=(
GEOMETRIC_REPRESENTATION_CONTEXT(3)
GLOBAL_UNCERTAINTY_ASSIGNED_CONTEXT((#2261))
GLOBAL_UNIT_ASSIGNED_CONTEXT((#2278,#2280,#2281))
REPRESENTATION_CONTEXT('','3D')
);
#2277=(
GEOMETRIC_REPRESENTATION_CONTEXT(3)
GLOBAL_UNCERTAINTY_ASSIGNED_CONTEXT((#2267))
GLOBAL_UNIT_ASSIGNED_CONTEXT((#2278,#2280,#2281))
REPRESENTATION_CONTEXT('','3D')
);
#2278=(
LENGTH_UNIT()
NAMED_UNIT(*)
SI_UNIT(.CENTI.,.METRE.)
);
#2280=(
NAMED_UNIT(*)
PLANE_ANGLE_UNIT()
SI_UNIT($,.RADIAN.)
);
#2281=(
NAMED_UNIT(*)
SI_UNIT($,.STERADIAN.)
SOLID_ANGLE_UNIT()
);
#2285=SHAPE_DEFINITION_REPRESENTATION(#2294,#2321);
#2294=PRODUCT_DEFINITION_SHAPE('',$,#2331);
#2321=SHAPE_REPRESENTATION('',(#1369),#2271);
#2327=PRODUCT_DEFINITION_CONTEXT('part definition',#2356,'design');
#2331=PRODUCT_DEFINITION('Housing','Housing',#2340,#2327);
#2340=PRODUCT_DEFINITION_FORMATION('',$,#2361);
#2356=APPLICATION_CONTEXT(
'Core Data for Automotive Mechanical Design Process');
#2357=PRODUCT_CONTEXT('part definition',#2356,'mechanical');
#2361=PRODUCT('Housing','Housing','Housing',(#2357));
#2368=PRESENTATION_STYLE_ASSIGNMENT((#2373));
#2373=SURFACE_STYLE_USAGE(.BOTH.,#2378);
#2378=SURFACE_SIDE_STYLE('',(#2383));
#2383=SURFACE_STYLE_FILL_AREA(#2388);
#2388=FILL_AREA_STYLE('Opaque(20,51,87)',(#2393));
#2393=FILL_AREA_STYLE_COLOUR('Opaque(20,51,87)',#2398);
#2398=COLOUR_RGB('Opaque(20,51,87)',0.0784313725490196,0.2,0.341176470588235);
ENDSEC;
END-ISO-10303-21;
